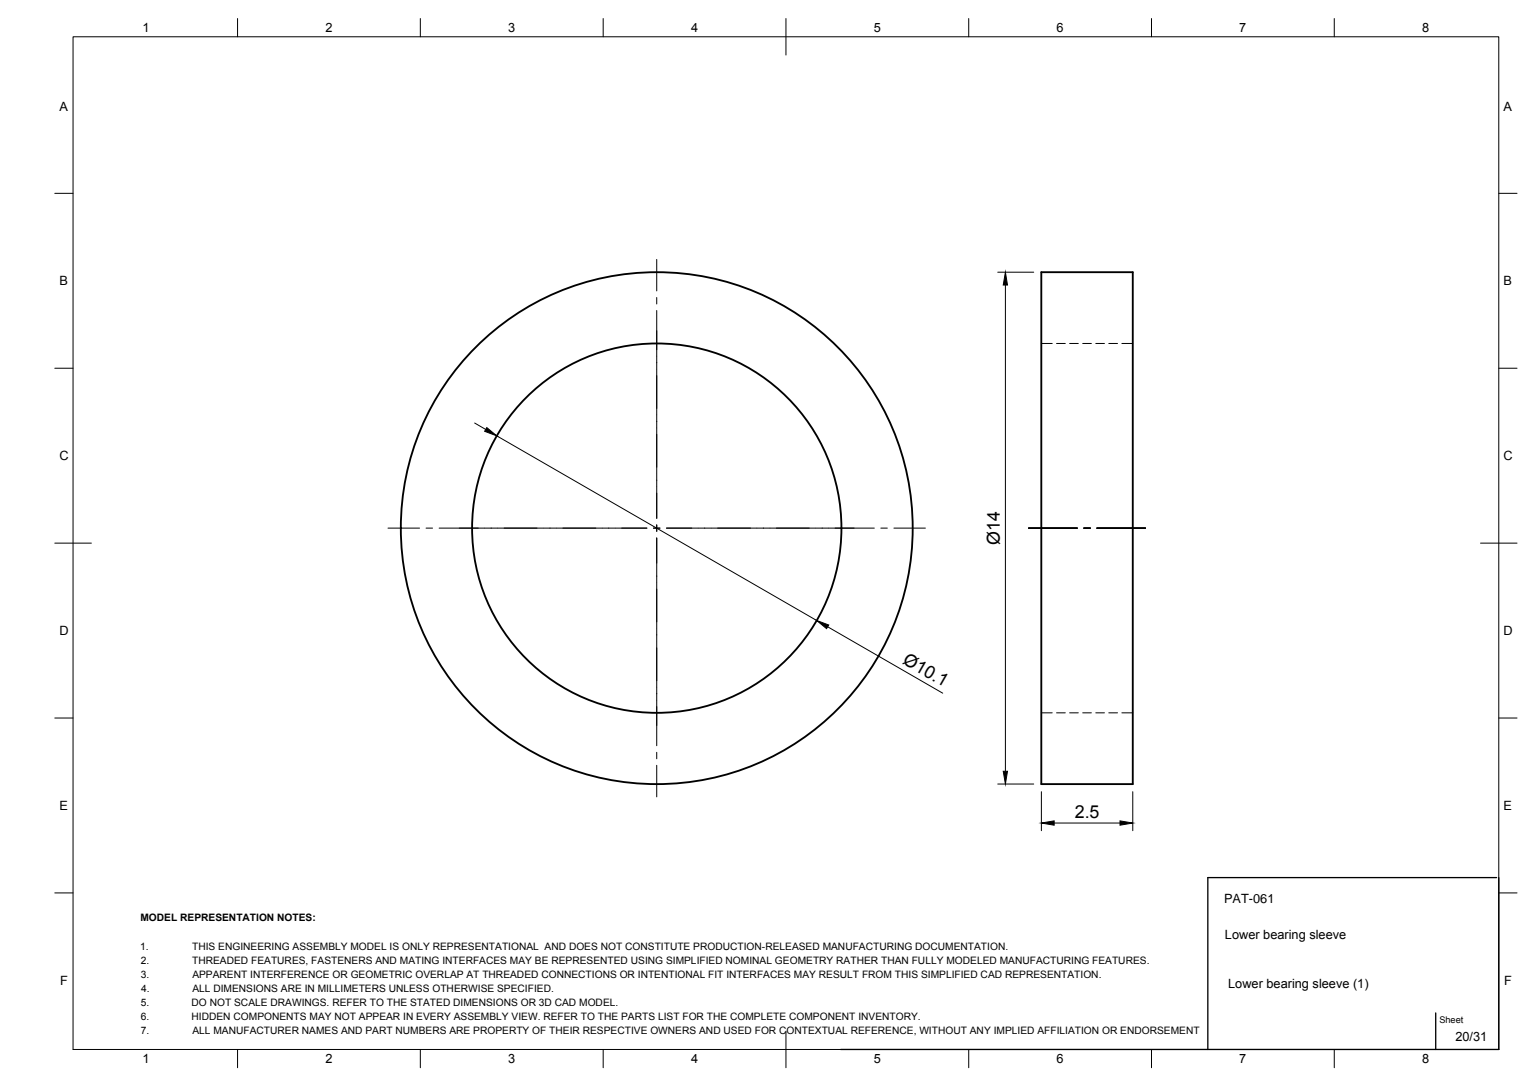
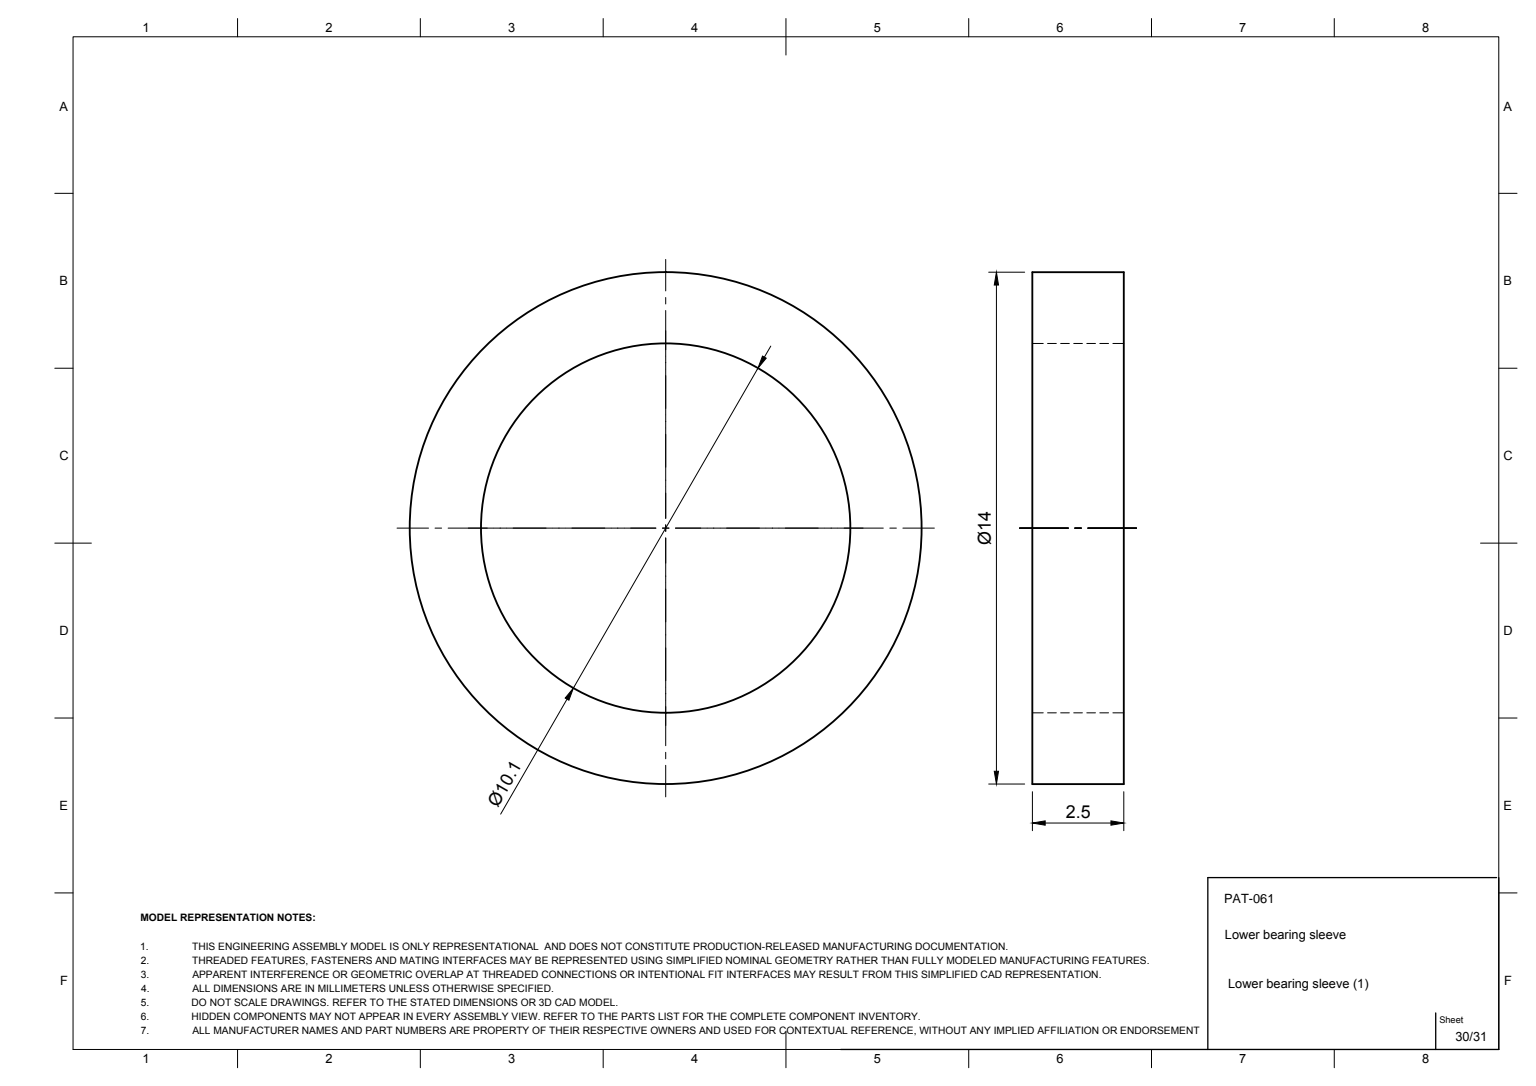
ISO-10303-21;
HEADER;
/* Generated by software containing ST-Developer
 * from STEP Tools, Inc. (www.steptools.com) 
 */

FILE_DESCRIPTION(
/* description */ ('Compact intermittent indexer'),
/* implementation_level */ '2;1');

FILE_NAME(
/* name */ 'Lower bearing sleeve.step',
/* time_stamp */ '2026-10-29T16:32:17-07:00',
/* author */ (''),
/* organization */ (''),
/* preprocessor_version */ 'ST-DEVELOPER v20.2',
/* originating_system */ 'Autodesk Translation Framework v15.17.0.0',
/* authorisation */ '');

FILE_SCHEMA (('AUTOMOTIVE_DESIGN { 1 0 10303 214 3 1 1 }'));
ENDSEC;

DATA;
#10=MECHANICAL_DESIGN_GEOMETRIC_PRESENTATION_REPRESENTATION('',(#277),#10837);
#221=SHAPE_REPRESENTATION_RELATIONSHIP('SRR','None',#10957,#245);
#245=ADVANCED_BREP_SHAPE_REPRESENTATION('',(#308),#10824);
#277=STYLED_ITEM('',(#11166),#308);
#308=MANIFOLD_SOLID_BREP('Body1',#5650);
#438=FACE_BOUND('',#1264,.T.);
#439=FACE_BOUND('',#1266,.T.);
#567=PLANE('',#6366);
#568=PLANE('',#6367);
#848=FACE_OUTER_BOUND('',#1261,.T.);
#849=FACE_OUTER_BOUND('',#1262,.T.);
#850=FACE_OUTER_BOUND('',#1263,.T.);
#851=FACE_OUTER_BOUND('',#1265,.T.);
#1261=EDGE_LOOP('',(#4518,#4519,#4520,#4521));
#1262=EDGE_LOOP('',(#4522,#4523,#4524,#4525));
#1263=EDGE_LOOP('',(#4526));
#1264=EDGE_LOOP('',(#4527));
#1265=EDGE_LOOP('',(#4528));
#1266=EDGE_LOOP('',(#4529));
#1603=LINE('',#9809,#1961);
#1604=LINE('',#9815,#1962);
#1961=VECTOR('',#7705,0.505);
#1962=VECTOR('',#7712,0.7);
#2362=CIRCLE('',#6361,0.505);
#2363=CIRCLE('',#6362,0.505);
#2364=CIRCLE('',#6364,0.7);
#2365=CIRCLE('',#6365,0.7);
#2760=VERTEX_POINT('',#9806);
#2761=VERTEX_POINT('',#9808);
#2762=VERTEX_POINT('',#9812);
#2763=VERTEX_POINT('',#9814);
#3381=EDGE_CURVE('',#2760,#2760,#2362,.T.);
#3382=EDGE_CURVE('',#2760,#2761,#1603,.T.);
#3383=EDGE_CURVE('',#2761,#2761,#2363,.T.);
#3384=EDGE_CURVE('',#2762,#2762,#2364,.T.);
#3385=EDGE_CURVE('',#2762,#2763,#1604,.T.);
#3386=EDGE_CURVE('',#2763,#2763,#2365,.T.);
#4518=ORIENTED_EDGE('',*,*,#3381,.F.);
#4519=ORIENTED_EDGE('',*,*,#3382,.T.);
#4520=ORIENTED_EDGE('',*,*,#3383,.T.);
#4521=ORIENTED_EDGE('',*,*,#3382,.F.);
#4522=ORIENTED_EDGE('',*,*,#3384,.F.);
#4523=ORIENTED_EDGE('',*,*,#3385,.T.);
#4524=ORIENTED_EDGE('',*,*,#3386,.T.);
#4525=ORIENTED_EDGE('',*,*,#3385,.F.);
#4526=ORIENTED_EDGE('',*,*,#3384,.T.);
#4527=ORIENTED_EDGE('',*,*,#3381,.T.);
#4528=ORIENTED_EDGE('',*,*,#3386,.F.);
#4529=ORIENTED_EDGE('',*,*,#3383,.F.);
#5246=CYLINDRICAL_SURFACE('',#6360,0.505);
#5247=CYLINDRICAL_SURFACE('',#6363,0.7);
#5491=ADVANCED_FACE('',(#848),#5246,.F.);
#5492=ADVANCED_FACE('',(#849),#5247,.T.);
#5493=ADVANCED_FACE('',(#850,#438),#567,.T.);
#5494=ADVANCED_FACE('',(#851,#439),#568,.F.);
#5650=CLOSED_SHELL('',(#5491,#5492,#5493,#5494));
#6359=AXIS2_PLACEMENT_3D('',#9804,#7699,#7700);
#6360=AXIS2_PLACEMENT_3D('',#9805,#7701,#7702);
#6361=AXIS2_PLACEMENT_3D('',#9807,#7703,#7704);
#6362=AXIS2_PLACEMENT_3D('',#9810,#7706,#7707);
#6363=AXIS2_PLACEMENT_3D('',#9811,#7708,#7709);
#6364=AXIS2_PLACEMENT_3D('',#9813,#7710,#7711);
#6365=AXIS2_PLACEMENT_3D('',#9816,#7713,#7714);
#6366=AXIS2_PLACEMENT_3D('',#9817,#7715,#7716);
#6367=AXIS2_PLACEMENT_3D('',#9818,#7717,#7718);
#7699=DIRECTION('axis',(0.,0.,1.));
#7700=DIRECTION('refdir',(1.,0.,0.));
#7701=DIRECTION('center_axis',(0.,0.,1.));
#7702=DIRECTION('ref_axis',(1.,0.,0.));
#7703=DIRECTION('center_axis',(0.,0.,-1.));
#7704=DIRECTION('ref_axis',(1.,0.,0.));
#7705=DIRECTION('',(0.,0.,-1.));
#7706=DIRECTION('center_axis',(0.,0.,-1.));
#7707=DIRECTION('ref_axis',(1.,0.,0.));
#7708=DIRECTION('center_axis',(0.,0.,1.));
#7709=DIRECTION('ref_axis',(1.,0.,0.));
#7710=DIRECTION('center_axis',(0.,0.,1.));
#7711=DIRECTION('ref_axis',(1.,0.,0.));
#7712=DIRECTION('',(0.,0.,-1.));
#7713=DIRECTION('center_axis',(0.,0.,1.));
#7714=DIRECTION('ref_axis',(1.,0.,0.));
#7715=DIRECTION('center_axis',(0.,0.,1.));
#7716=DIRECTION('ref_axis',(1.,0.,0.));
#7717=DIRECTION('center_axis',(0.,0.,1.));
#7718=DIRECTION('ref_axis',(1.,0.,0.));
#9804=CARTESIAN_POINT('',(0.,0.,0.));
#9805=CARTESIAN_POINT('Origin',(0.,0.,1.8));
#9806=CARTESIAN_POINT('',(-0.505,-6.18446633569413E-17,2.05));
#9807=CARTESIAN_POINT('Origin',(0.,0.,2.05));
#9808=CARTESIAN_POINT('',(-0.505,-6.18446633569413E-17,1.8));
#9809=CARTESIAN_POINT('',(-0.505,-6.18446633569413E-17,1.8));
#9810=CARTESIAN_POINT('Origin',(0.,0.,1.8));
#9811=CARTESIAN_POINT('Origin',(0.,0.,1.8));
#9812=CARTESIAN_POINT('',(-0.7,-8.57252759403147E-17,2.05));
#9813=CARTESIAN_POINT('Origin',(0.,0.,2.05));
#9814=CARTESIAN_POINT('',(-0.7,-8.57252759403147E-17,1.8));
#9815=CARTESIAN_POINT('',(-0.7,-8.57252759403147E-17,1.8));
#9816=CARTESIAN_POINT('Origin',(0.,0.,1.8));
#9817=CARTESIAN_POINT('Origin',(0.,0.,2.05));
#9818=CARTESIAN_POINT('Origin',(0.,0.,1.8));
#10794=UNCERTAINTY_MEASURE_WITH_UNIT(LENGTH_MEASURE(0.001),#10838,
'DISTANCE_ACCURACY_VALUE',
'Maximum model space distance between geometric entities at asserted c
onnectivities');
#10807=UNCERTAINTY_MEASURE_WITH_UNIT(LENGTH_MEASURE(0.001),#10838,
'DISTANCE_ACCURACY_VALUE',
'Maximum model space distance between geometric entities at asserted c
onnectivities');
#10824=(
GEOMETRIC_REPRESENTATION_CONTEXT(3)
GLOBAL_UNCERTAINTY_ASSIGNED_CONTEXT((#10794))
GLOBAL_UNIT_ASSIGNED_CONTEXT((#10838,#10840,#10841))
REPRESENTATION_CONTEXT('','3D')
);
#10837=(
GEOMETRIC_REPRESENTATION_CONTEXT(3)
GLOBAL_UNCERTAINTY_ASSIGNED_CONTEXT((#10807))
GLOBAL_UNIT_ASSIGNED_CONTEXT((#10838,#10840,#10841))
REPRESENTATION_CONTEXT('','3D')
);
#10838=(
LENGTH_UNIT()
NAMED_UNIT(*)
SI_UNIT(.CENTI.,.METRE.)
);
#10840=(
NAMED_UNIT(*)
PLANE_ANGLE_UNIT()
SI_UNIT($,.RADIAN.)
);
#10841=(
NAMED_UNIT(*)
SI_UNIT($,.STERADIAN.)
SOLID_ANGLE_UNIT()
);
#10858=SHAPE_DEFINITION_REPRESENTATION(#10892,#10957);
#10892=PRODUCT_DEFINITION_SHAPE('',$,#10987);
#10957=SHAPE_REPRESENTATION('',(#6359),#10824);
#10970=PRODUCT_DEFINITION_CONTEXT('part definition',#11059,'design');
#10987=PRODUCT_DEFINITION('Lower bearing sleeve','Lower bearing sleeve',
#11016,#10970);
#11016=PRODUCT_DEFINITION_FORMATION('',$,#11077);
#11059=APPLICATION_CONTEXT(
'Core Data for Automotive Mechanical Design Process');
#11060=PRODUCT_CONTEXT('part definition',#11059,'mechanical');
#11077=PRODUCT('Lower bearing sleeve','Lower bearing sleeve',
'Lower bearing sleeve',(#11060));
#11160=COLOUR_RGB('Grey',0.48,0.52,0.57);
#11161=FILL_AREA_STYLE_COLOUR('',#11160);
#11162=FILL_AREA_STYLE('',(#11161));
#11163=SURFACE_STYLE_FILL_AREA(#11162);
#11164=SURFACE_SIDE_STYLE('',(#11163));
#11165=SURFACE_STYLE_USAGE(.BOTH.,#11164);
#11166=PRESENTATION_STYLE_ASSIGNMENT((#11165));
ENDSEC;
END-ISO-10303-21;
